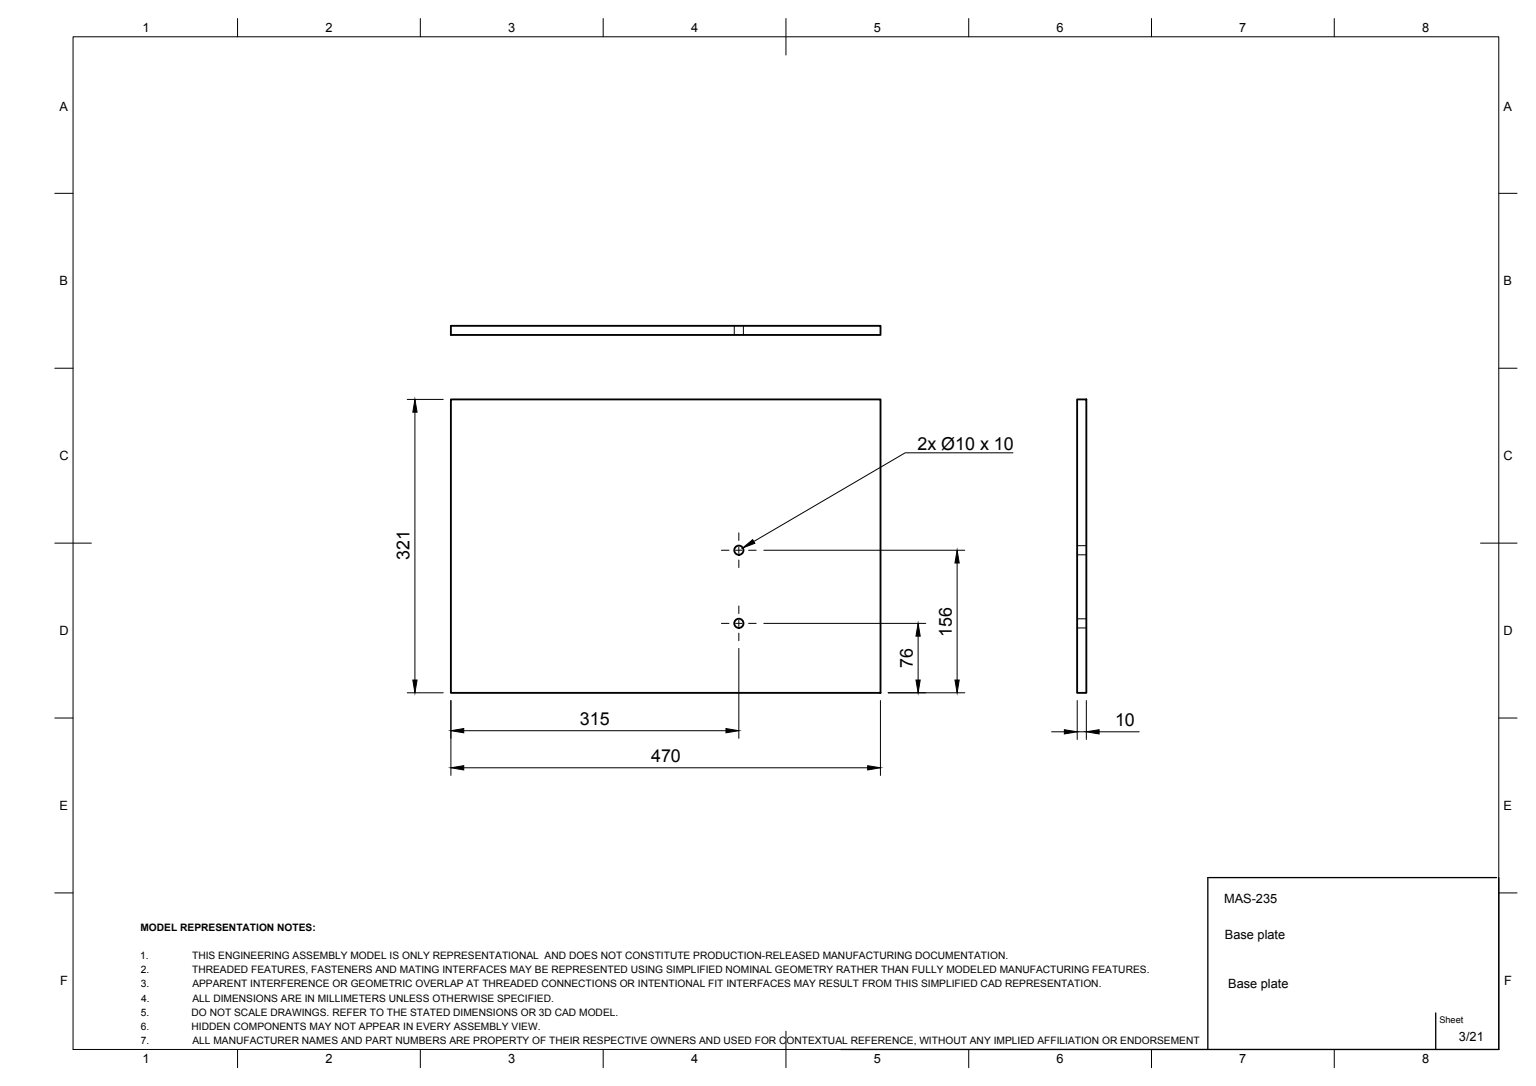
ISO-10303-21;
HEADER;
/* Generated by software containing ST-Developer
 * from STEP Tools, Inc. (www.steptools.com) 
 */

FILE_DESCRIPTION(
/* description */ ('Independent Whitworth quick-return mechanism. Crank radius40, ground-
center spacing80, lever180, connecting rod160, output guide X200. Nomi
nal stroke180 and long/short phase ratio2. Retained guide rods, replac
eable bearing sleeves and captured sliding shoe. No load or production
 rating assigned.'),
/* implementation_level */ '2;1');

FILE_NAME(
/* name */ 'Base plate.step',
/* time_stamp */ '2026-11-09T18:22:56-08:00',
/* author */ (''),
/* organization */ (''),
/* preprocessor_version */ 'ST-DEVELOPER v20.2',
/* originating_system */ 'Autodesk Translation Framework v15.17.0.0',
/* authorisation */ '');

FILE_SCHEMA (('AUTOMOTIVE_DESIGN { 1 0 10303 214 3 1 1 }'));
ENDSEC;

DATA;
#10=MECHANICAL_DESIGN_GEOMETRIC_PRESENTATION_REPRESENTATION('',(#219),#4388);
#179=SHAPE_REPRESENTATION_RELATIONSHIP('SRR','None',#4478,#199);
#199=ADVANCED_BREP_SHAPE_REPRESENTATION('',(#239),#4368);
#219=STYLED_ITEM('',(#4587),#239);
#239=MANIFOLD_SOLID_BREP('Body1',#2324);
#259=FACE_BOUND('',#559,.T.);
#260=FACE_BOUND('',#560,.T.);
#261=FACE_BOUND('',#562,.T.);
#262=FACE_BOUND('',#563,.T.);
#319=PLANE('',#2573);
#320=PLANE('',#2574);
#321=PLANE('',#2575);
#322=PLANE('',#2576);
#323=PLANE('',#2577);
#324=PLANE('',#2578);
#405=FACE_OUTER_BOUND('',#552,.T.);
#406=FACE_OUTER_BOUND('',#553,.T.);
#407=FACE_OUTER_BOUND('',#554,.T.);
#408=FACE_OUTER_BOUND('',#555,.T.);
#409=FACE_OUTER_BOUND('',#556,.T.);
#410=FACE_OUTER_BOUND('',#557,.T.);
#411=FACE_OUTER_BOUND('',#558,.T.);
#412=FACE_OUTER_BOUND('',#561,.T.);
#552=EDGE_LOOP('',(#1594,#1595,#1596,#1597));
#553=EDGE_LOOP('',(#1598,#1599,#1600,#1601));
#554=EDGE_LOOP('',(#1602,#1603,#1604,#1605));
#555=EDGE_LOOP('',(#1606,#1607,#1608,#1609));
#556=EDGE_LOOP('',(#1610,#1611,#1612,#1613));
#557=EDGE_LOOP('',(#1614,#1615,#1616,#1617));
#558=EDGE_LOOP('',(#1618,#1619,#1620,#1621));
#559=EDGE_LOOP('',(#1622));
#560=EDGE_LOOP('',(#1623));
#561=EDGE_LOOP('',(#1624,#1625,#1626,#1627));
#562=EDGE_LOOP('',(#1628));
#563=EDGE_LOOP('',(#1629));
#759=LINE('',#3706,#898);
#760=LINE('',#3712,#899);
#761=LINE('',#3717,#900);
#762=LINE('',#3719,#901);
#763=LINE('',#3721,#902);
#764=LINE('',#3722,#903);
#765=LINE('',#3725,#904);
#766=LINE('',#3727,#905);
#767=LINE('',#3728,#906);
#768=LINE('',#3731,#907);
#769=LINE('',#3733,#908);
#770=LINE('',#3734,#909);
#771=LINE('',#3736,#910);
#772=LINE('',#3737,#911);
#898=VECTOR('',#2905,5.);
#899=VECTOR('',#2912,5.);
#900=VECTOR('',#2917,10.);
#901=VECTOR('',#2918,10.);
#902=VECTOR('',#2919,10.);
#903=VECTOR('',#2920,10.);
#904=VECTOR('',#2923,10.);
#905=VECTOR('',#2924,10.);
#906=VECTOR('',#2925,10.);
#907=VECTOR('',#2928,10.);
#908=VECTOR('',#2929,10.);
#909=VECTOR('',#2930,10.);
#910=VECTOR('',#2933,10.);
#911=VECTOR('',#2934,10.);
#1037=CIRCLE('',#2568,5.);
#1038=CIRCLE('',#2569,5.);
#1039=CIRCLE('',#2571,5.);
#1040=CIRCLE('',#2572,5.);
#1159=VERTEX_POINT('',#3703);
#1160=VERTEX_POINT('',#3705);
#1161=VERTEX_POINT('',#3709);
#1162=VERTEX_POINT('',#3711);
#1163=VERTEX_POINT('',#3715);
#1164=VERTEX_POINT('',#3716);
#1165=VERTEX_POINT('',#3718);
#1166=VERTEX_POINT('',#3720);
#1167=VERTEX_POINT('',#3724);
#1168=VERTEX_POINT('',#3726);
#1169=VERTEX_POINT('',#3730);
#1170=VERTEX_POINT('',#3732);
#1333=EDGE_CURVE('',#1159,#1159,#1037,.T.);
#1334=EDGE_CURVE('',#1159,#1160,#759,.T.);
#1335=EDGE_CURVE('',#1160,#1160,#1038,.T.);
#1336=EDGE_CURVE('',#1161,#1161,#1039,.T.);
#1337=EDGE_CURVE('',#1161,#1162,#760,.T.);
#1338=EDGE_CURVE('',#1162,#1162,#1040,.T.);
#1339=EDGE_CURVE('',#1163,#1164,#761,.F.);
#1340=EDGE_CURVE('',#1164,#1165,#762,.T.);
#1341=EDGE_CURVE('',#1166,#1165,#763,.F.);
#1342=EDGE_CURVE('',#1163,#1166,#764,.F.);
#1343=EDGE_CURVE('',#1167,#1163,#765,.F.);
#1344=EDGE_CURVE('',#1168,#1166,#766,.F.);
#1345=EDGE_CURVE('',#1167,#1168,#767,.F.);
#1346=EDGE_CURVE('',#1169,#1167,#768,.F.);
#1347=EDGE_CURVE('',#1170,#1168,#769,.F.);
#1348=EDGE_CURVE('',#1169,#1170,#770,.T.);
#1349=EDGE_CURVE('',#1164,#1169,#771,.F.);
#1350=EDGE_CURVE('',#1165,#1170,#772,.F.);
#1594=ORIENTED_EDGE('',*,*,#1333,.F.);
#1595=ORIENTED_EDGE('',*,*,#1334,.T.);
#1596=ORIENTED_EDGE('',*,*,#1335,.F.);
#1597=ORIENTED_EDGE('',*,*,#1334,.F.);
#1598=ORIENTED_EDGE('',*,*,#1336,.F.);
#1599=ORIENTED_EDGE('',*,*,#1337,.T.);
#1600=ORIENTED_EDGE('',*,*,#1338,.F.);
#1601=ORIENTED_EDGE('',*,*,#1337,.F.);
#1602=ORIENTED_EDGE('',*,*,#1339,.T.);
#1603=ORIENTED_EDGE('',*,*,#1340,.T.);
#1604=ORIENTED_EDGE('',*,*,#1341,.F.);
#1605=ORIENTED_EDGE('',*,*,#1342,.F.);
#1606=ORIENTED_EDGE('',*,*,#1343,.T.);
#1607=ORIENTED_EDGE('',*,*,#1342,.T.);
#1608=ORIENTED_EDGE('',*,*,#1344,.F.);
#1609=ORIENTED_EDGE('',*,*,#1345,.F.);
#1610=ORIENTED_EDGE('',*,*,#1346,.T.);
#1611=ORIENTED_EDGE('',*,*,#1345,.T.);
#1612=ORIENTED_EDGE('',*,*,#1347,.F.);
#1613=ORIENTED_EDGE('',*,*,#1348,.F.);
#1614=ORIENTED_EDGE('',*,*,#1349,.T.);
#1615=ORIENTED_EDGE('',*,*,#1348,.T.);
#1616=ORIENTED_EDGE('',*,*,#1350,.F.);
#1617=ORIENTED_EDGE('',*,*,#1340,.F.);
#1618=ORIENTED_EDGE('',*,*,#1350,.T.);
#1619=ORIENTED_EDGE('',*,*,#1347,.T.);
#1620=ORIENTED_EDGE('',*,*,#1344,.T.);
#1621=ORIENTED_EDGE('',*,*,#1341,.T.);
#1622=ORIENTED_EDGE('',*,*,#1333,.T.);
#1623=ORIENTED_EDGE('',*,*,#1336,.T.);
#1624=ORIENTED_EDGE('',*,*,#1349,.F.);
#1625=ORIENTED_EDGE('',*,*,#1339,.F.);
#1626=ORIENTED_EDGE('',*,*,#1343,.F.);
#1627=ORIENTED_EDGE('',*,*,#1346,.F.);
#1628=ORIENTED_EDGE('',*,*,#1335,.T.);
#1629=ORIENTED_EDGE('',*,*,#1338,.T.);
#2116=CYLINDRICAL_SURFACE('',#2567,5.);
#2117=CYLINDRICAL_SURFACE('',#2570,5.);
#2177=ADVANCED_FACE('',(#405),#2116,.F.);
#2178=ADVANCED_FACE('',(#406),#2117,.F.);
#2179=ADVANCED_FACE('',(#407),#319,.T.);
#2180=ADVANCED_FACE('',(#408),#320,.T.);
#2181=ADVANCED_FACE('',(#409),#321,.T.);
#2182=ADVANCED_FACE('',(#410),#322,.T.);
#2183=ADVANCED_FACE('',(#411,#259,#260),#323,.T.);
#2184=ADVANCED_FACE('',(#412,#261,#262),#324,.F.);
#2324=CLOSED_SHELL('',(#2177,#2178,#2179,#2180,#2181,#2182,#2183,#2184));
#2566=AXIS2_PLACEMENT_3D('',#3701,#2899,#2900);
#2567=AXIS2_PLACEMENT_3D('',#3702,#2901,#2902);
#2568=AXIS2_PLACEMENT_3D('',#3704,#2903,#2904);
#2569=AXIS2_PLACEMENT_3D('',#3707,#2906,#2907);
#2570=AXIS2_PLACEMENT_3D('',#3708,#2908,#2909);
#2571=AXIS2_PLACEMENT_3D('',#3710,#2910,#2911);
#2572=AXIS2_PLACEMENT_3D('',#3713,#2913,#2914);
#2573=AXIS2_PLACEMENT_3D('',#3714,#2915,#2916);
#2574=AXIS2_PLACEMENT_3D('',#3723,#2921,#2922);
#2575=AXIS2_PLACEMENT_3D('',#3729,#2926,#2927);
#2576=AXIS2_PLACEMENT_3D('',#3735,#2931,#2932);
#2577=AXIS2_PLACEMENT_3D('',#3738,#2935,#2936);
#2578=AXIS2_PLACEMENT_3D('',#3739,#2937,#2938);
#2899=DIRECTION('axis',(0.,0.,1.));
#2900=DIRECTION('refdir',(1.,0.,0.));
#2901=DIRECTION('center_axis',(0.,0.,-1.));
#2902=DIRECTION('ref_axis',(1.,0.,0.));
#2903=DIRECTION('center_axis',(0.,0.,-1.));
#2904=DIRECTION('ref_axis',(1.,0.,0.));
#2905=DIRECTION('',(0.,0.,-1.));
#2906=DIRECTION('center_axis',(0.,0.,1.));
#2907=DIRECTION('ref_axis',(1.,0.,0.));
#2908=DIRECTION('center_axis',(0.,0.,-1.));
#2909=DIRECTION('ref_axis',(1.,0.,0.));
#2910=DIRECTION('center_axis',(0.,0.,-1.));
#2911=DIRECTION('ref_axis',(1.,0.,0.));
#2912=DIRECTION('',(0.,0.,-1.));
#2913=DIRECTION('center_axis',(0.,0.,1.));
#2914=DIRECTION('ref_axis',(1.,0.,0.));
#2915=DIRECTION('center_axis',(0.,1.,0.));
#2916=DIRECTION('ref_axis',(-1.,0.,0.));
#2917=DIRECTION('',(1.,0.,0.));
#2918=DIRECTION('',(0.,0.,1.));
#2919=DIRECTION('',(1.,0.,0.));
#2920=DIRECTION('',(0.,0.,-1.));
#2921=DIRECTION('center_axis',(1.,0.,0.));
#2922=DIRECTION('ref_axis',(0.,1.,0.));
#2923=DIRECTION('',(0.,-1.,0.));
#2924=DIRECTION('',(0.,-1.,0.));
#2925=DIRECTION('',(0.,0.,-1.));
#2926=DIRECTION('center_axis',(0.,-1.,0.));
#2927=DIRECTION('ref_axis',(1.,0.,0.));
#2928=DIRECTION('',(-1.,0.,0.));
#2929=DIRECTION('',(-1.,0.,0.));
#2930=DIRECTION('',(0.,0.,1.));
#2931=DIRECTION('center_axis',(-1.,0.,0.));
#2932=DIRECTION('ref_axis',(0.,-1.,0.));
#2933=DIRECTION('',(0.,1.,0.));
#2934=DIRECTION('',(0.,1.,0.));
#2935=DIRECTION('center_axis',(0.,0.,1.));
#2936=DIRECTION('ref_axis',(1.,0.,0.));
#2937=DIRECTION('center_axis',(0.,0.,1.));
#2938=DIRECTION('ref_axis',(1.,0.,0.));
#3701=CARTESIAN_POINT('',(0.,0.,0.));
#3702=CARTESIAN_POINT('Origin',(0.,0.,5.));
#3703=CARTESIAN_POINT('',(-5.,6.12323399573677E-16,10.));
#3704=CARTESIAN_POINT('Origin',(0.,0.,10.));
#3705=CARTESIAN_POINT('',(-5.,6.12323399573677E-16,0.));
#3706=CARTESIAN_POINT('',(-5.,6.12323399573677E-16,5.));
#3707=CARTESIAN_POINT('Origin',(0.,0.,0.));
#3708=CARTESIAN_POINT('Origin',(80.,0.,5.));
#3709=CARTESIAN_POINT('',(75.,6.12323399573677E-16,10.));
#3710=CARTESIAN_POINT('Origin',(80.,0.,10.));
#3711=CARTESIAN_POINT('',(75.,6.12323399573677E-16,0.));
#3712=CARTESIAN_POINT('',(75.,6.12323399573677E-16,5.));
#3713=CARTESIAN_POINT('Origin',(80.,0.,0.));
#3714=CARTESIAN_POINT('Origin',(240.,315.,0.));
#3715=CARTESIAN_POINT('',(245.,315.,0.));
#3716=CARTESIAN_POINT('',(-76.,315.,0.));
#3717=CARTESIAN_POINT('',(160.,315.,0.));
#3718=CARTESIAN_POINT('',(-76.,315.,10.));
#3719=CARTESIAN_POINT('',(-76.,315.,0.));
#3720=CARTESIAN_POINT('',(245.,315.,10.));
#3721=CARTESIAN_POINT('',(160.,315.,10.));
#3722=CARTESIAN_POINT('',(245.,315.,0.));
#3723=CARTESIAN_POINT('Origin',(245.,-150.,0.));
#3724=CARTESIAN_POINT('',(245.,-155.,0.));
#3725=CARTESIAN_POINT('',(245.,-35.,0.));
#3726=CARTESIAN_POINT('',(245.,-155.,10.));
#3727=CARTESIAN_POINT('',(245.,-35.,10.));
#3728=CARTESIAN_POINT('',(245.,-155.,0.));
#3729=CARTESIAN_POINT('Origin',(-80.,-155.,0.));
#3730=CARTESIAN_POINT('',(-76.,-155.,0.));
#3731=CARTESIAN_POINT('',(0.,-155.,0.));
#3732=CARTESIAN_POINT('',(-76.,-155.,10.));
#3733=CARTESIAN_POINT('',(0.,-155.,10.));
#3734=CARTESIAN_POINT('',(-76.,-155.,0.));
#3735=CARTESIAN_POINT('Origin',(-76.,310.,0.));
#3736=CARTESIAN_POINT('',(-76.,195.,0.));
#3737=CARTESIAN_POINT('',(-76.,195.,10.));
#3738=CARTESIAN_POINT('Origin',(80.,80.,10.));
#3739=CARTESIAN_POINT('Origin',(80.,80.,0.));
#4346=UNCERTAINTY_MEASURE_WITH_UNIT(LENGTH_MEASURE(0.01),#4389,
'DISTANCE_ACCURACY_VALUE',
'Maximum model space distance between geometric entities at asserted c
onnectivities');
#4366=UNCERTAINTY_MEASURE_WITH_UNIT(LENGTH_MEASURE(0.01),#4389,
'DISTANCE_ACCURACY_VALUE',
'Maximum model space distance between geometric entities at asserted c
onnectivities');
#4368=(
GEOMETRIC_REPRESENTATION_CONTEXT(3)
GLOBAL_UNCERTAINTY_ASSIGNED_CONTEXT((#4346))
GLOBAL_UNIT_ASSIGNED_CONTEXT((#4389,#4391,#4392))
REPRESENTATION_CONTEXT('','3D')
);
#4388=(
GEOMETRIC_REPRESENTATION_CONTEXT(3)
GLOBAL_UNCERTAINTY_ASSIGNED_CONTEXT((#4366))
GLOBAL_UNIT_ASSIGNED_CONTEXT((#4389,#4391,#4392))
REPRESENTATION_CONTEXT('','3D')
);
#4389=(
LENGTH_UNIT()
NAMED_UNIT(*)
SI_UNIT(.MILLI.,.METRE.)
);
#4391=(
NAMED_UNIT(*)
PLANE_ANGLE_UNIT()
SI_UNIT($,.RADIAN.)
);
#4392=(
NAMED_UNIT(*)
SI_UNIT($,.STERADIAN.)
SOLID_ANGLE_UNIT()
);
#4394=SHAPE_DEFINITION_REPRESENTATION(#4415,#4478);
#4415=PRODUCT_DEFINITION_SHAPE('',$,#4500);
#4478=SHAPE_REPRESENTATION('',(#2566),#4368);
#4498=PRODUCT_DEFINITION_CONTEXT('part definition',#4563,'design');
#4500=PRODUCT_DEFINITION('Base plate','Base plate',#4521,#4498);
#4521=PRODUCT_DEFINITION_FORMATION('',$,#4566);
#4563=APPLICATION_CONTEXT(
'Core Data for Automotive Mechanical Design Process');
#4564=PRODUCT_CONTEXT('part definition',#4563,'mechanical');
#4566=PRODUCT('Base plate','Base plate','Base plate',(#4564));
#4587=PRESENTATION_STYLE_ASSIGNMENT((#4601));
#4601=SURFACE_STYLE_USAGE(.BOTH.,#4615);
#4615=SURFACE_SIDE_STYLE('',(#4629));
#4629=SURFACE_STYLE_FILL_AREA(#4643);
#4643=FILL_AREA_STYLE('Base gray',(#4657));
#4657=FILL_AREA_STYLE_COLOUR('Base gray',#4671);
#4671=COLOUR_RGB('Base gray',0.407843137254902,0.447058823529412,0.498039215686275);
ENDSEC;
END-ISO-10303-21;
